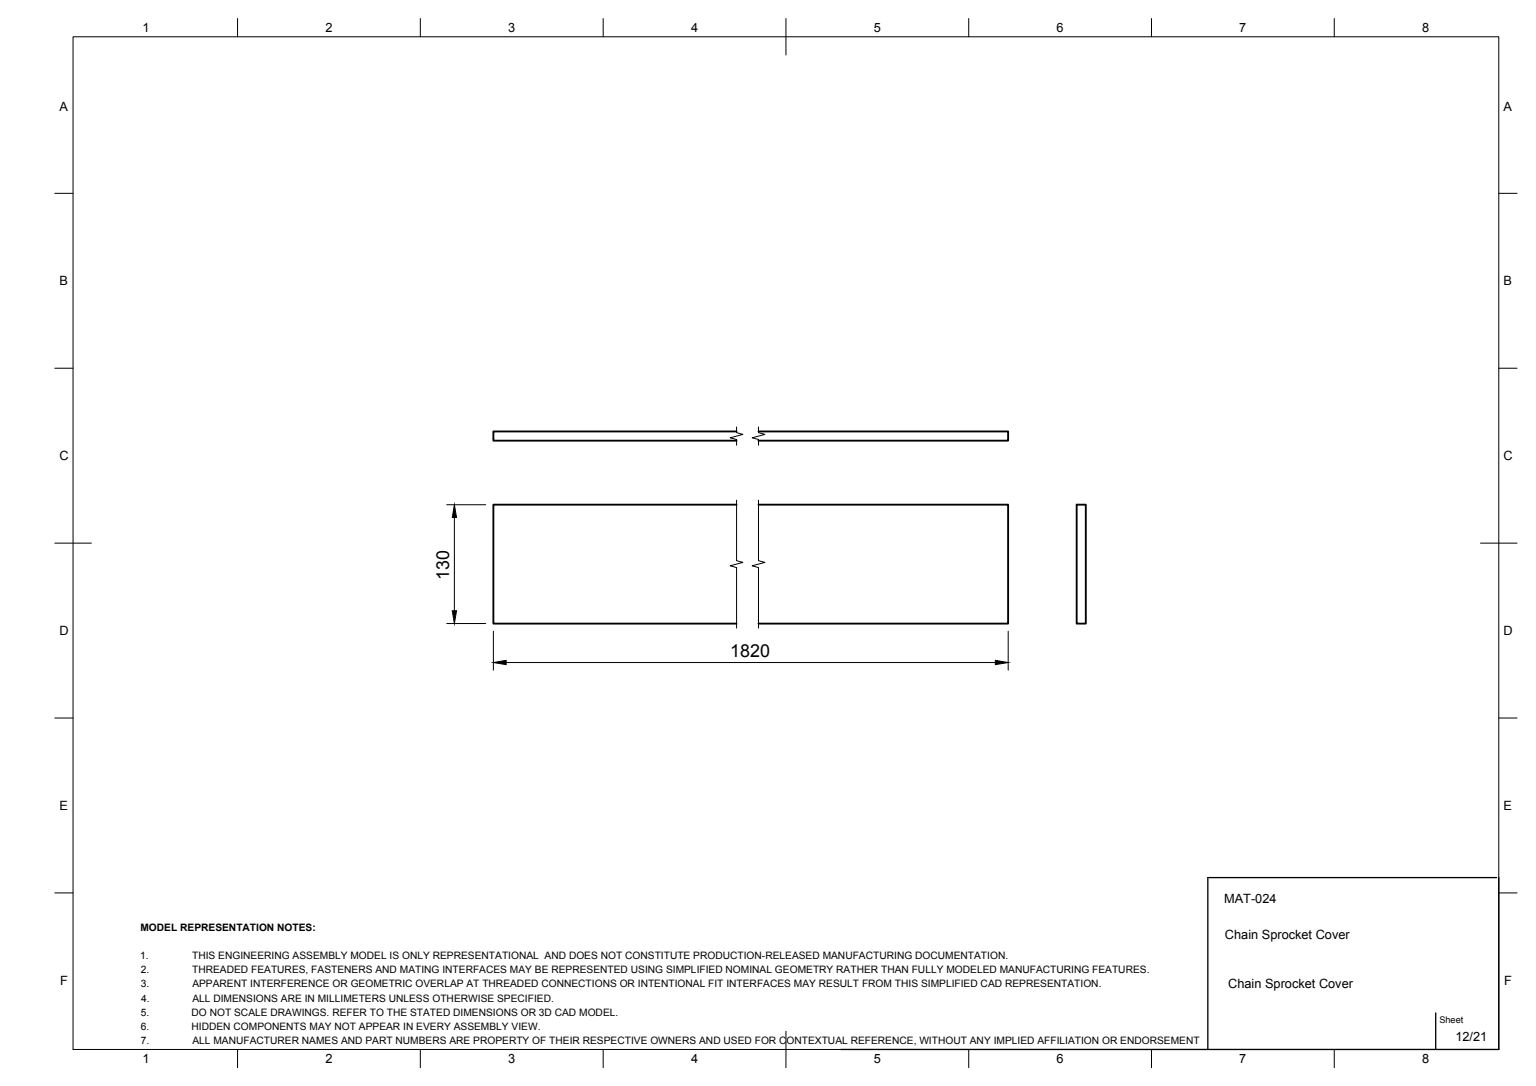
ISO-10303-21;
HEADER;
/* Generated by software containing ST-Developer
 * from STEP Tools, Inc. (www.steptools.com) 
 */

FILE_DESCRIPTION(
/* description */ ('STEP AP214'),
/* implementation_level */ '2;1');

FILE_NAME(
/* name */ 'Chain Sprocket Cover.step',
/* time_stamp */ '2026-11-14T06:34:07-08:00',
/* author */ (''),
/* organization */ (''),
/* preprocessor_version */ 'ST-DEVELOPER v20.2',
/* originating_system */ 'Autodesk Translation Framework v15.17.0.0',
/* authorisation */ '');

FILE_SCHEMA (('AUTOMOTIVE_DESIGN { 1 0 10303 214 3 1 1 }'));
ENDSEC;

DATA;
#10=MECHANICAL_DESIGN_GEOMETRIC_PRESENTATION_REPRESENTATION('',(#7278),#310623);
#7225=SHAPE_REPRESENTATION_RELATIONSHIP('SRR','None',#310897,#7242);
#7242=ADVANCED_BREP_SHAPE_REPRESENTATION('',(#7346),#310606);
#7278=STYLED_ITEM('',(#311006),#7346);
#7346=MANIFOLD_SOLID_BREP('Body1',#93728);
#8518=PLANE('',#103333);
#8519=PLANE('',#103334);
#8520=PLANE('',#103335);
#8521=PLANE('',#103336);
#8522=PLANE('',#103337);
#8523=PLANE('',#103338);
#13629=FACE_OUTER_BOUND('',#19599,.T.);
#13630=FACE_OUTER_BOUND('',#19600,.T.);
#13631=FACE_OUTER_BOUND('',#19601,.T.);
#13632=FACE_OUTER_BOUND('',#19602,.T.);
#13633=FACE_OUTER_BOUND('',#19603,.T.);
#13634=FACE_OUTER_BOUND('',#19604,.T.);
#19599=EDGE_LOOP('',(#81693,#81694,#81695,#81696));
#19600=EDGE_LOOP('',(#81697,#81698,#81699,#81700));
#19601=EDGE_LOOP('',(#81701,#81702,#81703,#81704));
#19602=EDGE_LOOP('',(#81705,#81706,#81707,#81708));
#19603=EDGE_LOOP('',(#81709,#81710,#81711,#81712));
#19604=EDGE_LOOP('',(#81713,#81714,#81715,#81716));
#24192=LINE('',#271199,#28539);
#24193=LINE('',#271201,#28540);
#24194=LINE('',#271203,#28541);
#24195=LINE('',#271204,#28542);
#24196=LINE('',#271207,#28543);
#24197=LINE('',#271209,#28544);
#24198=LINE('',#271210,#28545);
#24199=LINE('',#271213,#28546);
#24200=LINE('',#271215,#28547);
#24201=LINE('',#271216,#28548);
#24202=LINE('',#271218,#28549);
#24203=LINE('',#271219,#28550);
#28539=VECTOR('',#127317,1000.);
#28540=VECTOR('',#127318,1000.);
#28541=VECTOR('',#127319,1000.);
#28542=VECTOR('',#127320,1000.);
#28543=VECTOR('',#127323,1000.);
#28544=VECTOR('',#127324,1000.);
#28545=VECTOR('',#127325,1000.);
#28546=VECTOR('',#127328,1000.);
#28547=VECTOR('',#127329,1000.);
#28548=VECTOR('',#127330,1000.);
#28549=VECTOR('',#127333,1000.);
#28550=VECTOR('',#127334,1000.);
#42245=VERTEX_POINT('',#271197);
#42246=VERTEX_POINT('',#271198);
#42247=VERTEX_POINT('',#271200);
#42248=VERTEX_POINT('',#271202);
#42249=VERTEX_POINT('',#271206);
#42250=VERTEX_POINT('',#271208);
#42251=VERTEX_POINT('',#271212);
#42252=VERTEX_POINT('',#271214);
#55626=EDGE_CURVE('',#42245,#42246,#24192,.T.);
#55627=EDGE_CURVE('',#42247,#42246,#24193,.T.);
#55628=EDGE_CURVE('',#42248,#42247,#24194,.T.);
#55629=EDGE_CURVE('',#42248,#42245,#24195,.T.);
#55630=EDGE_CURVE('',#42246,#42249,#24196,.T.);
#55631=EDGE_CURVE('',#42250,#42249,#24197,.T.);
#55632=EDGE_CURVE('',#42247,#42250,#24198,.T.);
#55633=EDGE_CURVE('',#42249,#42251,#24199,.T.);
#55634=EDGE_CURVE('',#42252,#42251,#24200,.T.);
#55635=EDGE_CURVE('',#42250,#42252,#24201,.T.);
#55636=EDGE_CURVE('',#42251,#42245,#24202,.T.);
#55637=EDGE_CURVE('',#42252,#42248,#24203,.T.);
#81693=ORIENTED_EDGE('',*,*,#55626,.T.);
#81694=ORIENTED_EDGE('',*,*,#55627,.F.);
#81695=ORIENTED_EDGE('',*,*,#55628,.F.);
#81696=ORIENTED_EDGE('',*,*,#55629,.T.);
#81697=ORIENTED_EDGE('',*,*,#55630,.T.);
#81698=ORIENTED_EDGE('',*,*,#55631,.F.);
#81699=ORIENTED_EDGE('',*,*,#55632,.F.);
#81700=ORIENTED_EDGE('',*,*,#55627,.T.);
#81701=ORIENTED_EDGE('',*,*,#55633,.T.);
#81702=ORIENTED_EDGE('',*,*,#55634,.F.);
#81703=ORIENTED_EDGE('',*,*,#55635,.F.);
#81704=ORIENTED_EDGE('',*,*,#55631,.T.);
#81705=ORIENTED_EDGE('',*,*,#55636,.T.);
#81706=ORIENTED_EDGE('',*,*,#55629,.F.);
#81707=ORIENTED_EDGE('',*,*,#55637,.F.);
#81708=ORIENTED_EDGE('',*,*,#55634,.T.);
#81709=ORIENTED_EDGE('',*,*,#55628,.T.);
#81710=ORIENTED_EDGE('',*,*,#55632,.T.);
#81711=ORIENTED_EDGE('',*,*,#55635,.T.);
#81712=ORIENTED_EDGE('',*,*,#55637,.T.);
#81713=ORIENTED_EDGE('',*,*,#55626,.F.);
#81714=ORIENTED_EDGE('',*,*,#55636,.F.);
#81715=ORIENTED_EDGE('',*,*,#55633,.F.);
#81716=ORIENTED_EDGE('',*,*,#55630,.F.);
#92908=ADVANCED_FACE('',(#13629),#8518,.F.);
#92909=ADVANCED_FACE('',(#13630),#8519,.F.);
#92910=ADVANCED_FACE('',(#13631),#8520,.F.);
#92911=ADVANCED_FACE('',(#13632),#8521,.F.);
#92912=ADVANCED_FACE('',(#13633),#8522,.T.);
#92913=ADVANCED_FACE('',(#13634),#8523,.F.);
#93728=CLOSED_SHELL('',(#92908,#92909,#92910,#92911,#92912,#92913));
#103332=AXIS2_PLACEMENT_3D('',#271195,#127313,#127314);
#103333=AXIS2_PLACEMENT_3D('',#271196,#127315,#127316);
#103334=AXIS2_PLACEMENT_3D('',#271205,#127321,#127322);
#103335=AXIS2_PLACEMENT_3D('',#271211,#127326,#127327);
#103336=AXIS2_PLACEMENT_3D('',#271217,#127331,#127332);
#103337=AXIS2_PLACEMENT_3D('',#271220,#127335,#127336);
#103338=AXIS2_PLACEMENT_3D('',#271221,#127337,#127338);
#127313=DIRECTION('axis',(0.,0.,1.));
#127314=DIRECTION('refdir',(1.,0.,0.));
#127315=DIRECTION('center_axis',(0.,0.,-1.));
#127316=DIRECTION('ref_axis',(-1.,0.,0.));
#127317=DIRECTION('',(0.,-1.,0.));
#127318=DIRECTION('',(-1.,0.,0.));
#127319=DIRECTION('',(0.,-1.,0.));
#127320=DIRECTION('',(-1.,0.,0.));
#127321=DIRECTION('center_axis',(0.,1.,1.52503162723236E-17));
#127322=DIRECTION('ref_axis',(0.,-1.52503162723236E-17,1.));
#127323=DIRECTION('',(0.,1.52503162723236E-17,-1.));
#127324=DIRECTION('',(-1.,0.,0.));
#127325=DIRECTION('',(0.,1.52503162723236E-17,-1.));
#127326=DIRECTION('center_axis',(0.,0.,1.));
#127327=DIRECTION('ref_axis',(1.,0.,0.));
#127328=DIRECTION('',(0.,1.,0.));
#127329=DIRECTION('',(-1.,0.,0.));
#127330=DIRECTION('',(0.,1.,0.));
#127331=DIRECTION('center_axis',(0.,-1.,0.));
#127332=DIRECTION('ref_axis',(0.,0.,-1.));
#127333=DIRECTION('',(0.,0.,1.));
#127334=DIRECTION('',(0.,0.,1.));
#127335=DIRECTION('center_axis',(1.,0.,0.));
#127336=DIRECTION('ref_axis',(0.,0.,-1.));
#127337=DIRECTION('center_axis',(1.,0.,0.));
#127338=DIRECTION('ref_axis',(0.,0.,-1.));
#271195=CARTESIAN_POINT('',(0.,0.,0.));
#271196=CARTESIAN_POINT('Origin',(10.,130.,910.));
#271197=CARTESIAN_POINT('',(0.,130.,910.));
#271198=CARTESIAN_POINT('',(0.,0.,910.));
#271199=CARTESIAN_POINT('',(0.,130.,910.));
#271200=CARTESIAN_POINT('',(10.,0.,910.));
#271201=CARTESIAN_POINT('',(10.,0.,910.));
#271202=CARTESIAN_POINT('',(10.,130.,910.));
#271203=CARTESIAN_POINT('',(10.,130.,910.));
#271204=CARTESIAN_POINT('',(10.,130.,910.));
#271205=CARTESIAN_POINT('Origin',(10.,0.,910.));
#271206=CARTESIAN_POINT('',(0.,2.77555756156289E-14,-910.));
#271207=CARTESIAN_POINT('',(0.,0.,910.));
#271208=CARTESIAN_POINT('',(10.,2.77555756156289E-14,-910.));
#271209=CARTESIAN_POINT('',(10.,2.77555756156289E-14,-910.));
#271210=CARTESIAN_POINT('',(10.,0.,910.));
#271211=CARTESIAN_POINT('Origin',(10.,130.,-910.));
#271212=CARTESIAN_POINT('',(0.,130.,-910.));
#271213=CARTESIAN_POINT('',(0.,130.,-910.));
#271214=CARTESIAN_POINT('',(10.,130.,-910.));
#271215=CARTESIAN_POINT('',(10.,130.,-910.));
#271216=CARTESIAN_POINT('',(10.,130.,-910.));
#271217=CARTESIAN_POINT('Origin',(10.,130.,910.));
#271218=CARTESIAN_POINT('',(0.,130.,910.));
#271219=CARTESIAN_POINT('',(10.,130.,910.));
#271220=CARTESIAN_POINT('Origin',(10.,0.,0.));
#271221=CARTESIAN_POINT('Origin',(0.,0.,0.));
#310584=UNCERTAINTY_MEASURE_WITH_UNIT(LENGTH_MEASURE(0.01),#310624,
'DISTANCE_ACCURACY_VALUE',
'Maximum model space distance between geometric entities at asserted c
onnectivities');
#310601=UNCERTAINTY_MEASURE_WITH_UNIT(LENGTH_MEASURE(0.01),#310624,
'DISTANCE_ACCURACY_VALUE',
'Maximum model space distance between geometric entities at asserted c
onnectivities');
#310606=(
GEOMETRIC_REPRESENTATION_CONTEXT(3)
GLOBAL_UNCERTAINTY_ASSIGNED_CONTEXT((#310584))
GLOBAL_UNIT_ASSIGNED_CONTEXT((#310624,#310626,#310627))
REPRESENTATION_CONTEXT('','3D')
);
#310623=(
GEOMETRIC_REPRESENTATION_CONTEXT(3)
GLOBAL_UNCERTAINTY_ASSIGNED_CONTEXT((#310601))
GLOBAL_UNIT_ASSIGNED_CONTEXT((#310624,#310626,#310627))
REPRESENTATION_CONTEXT('','3D')
);
#310624=(
LENGTH_UNIT()
NAMED_UNIT(*)
SI_UNIT(.MILLI.,.METRE.)
);
#310626=(
NAMED_UNIT(*)
PLANE_ANGLE_UNIT()
SI_UNIT($,.RADIAN.)
);
#310627=(
NAMED_UNIT(*)
SI_UNIT($,.STERADIAN.)
SOLID_ANGLE_UNIT()
);
#310632=SHAPE_DEFINITION_REPRESENTATION(#310653,#310897);
#310653=PRODUCT_DEFINITION_SHAPE('',$,#310919);
#310897=SHAPE_REPRESENTATION('',(#103332),#310606);
#310914=PRODUCT_DEFINITION_CONTEXT('part definition',#310979,'design');
#310919=PRODUCT_DEFINITION('Chain Sprocket Cover',
'Chain Sprocket Cover',#310940,#310914);
#310940=PRODUCT_DEFINITION_FORMATION('',$,#310985);
#310979=APPLICATION_CONTEXT(
'Core Data for Automotive Mechanical Design Process');
#310980=PRODUCT_CONTEXT('part definition',#310979,'mechanical');
#310985=PRODUCT('Chain Sprocket Cover','Chain Sprocket Cover',$,(#310980));
#311006=PRESENTATION_STYLE_ASSIGNMENT((#311013));
#311013=SURFACE_STYLE_USAGE(.BOTH.,#311020);
#311020=SURFACE_SIDE_STYLE('',(#311027));
#311027=SURFACE_STYLE_FILL_AREA(#311034);
#311034=FILL_AREA_STYLE('Opaque(61,176,222)',(#311041));
#311041=FILL_AREA_STYLE_COLOUR('Opaque(61,176,222)',#311048);
#311048=COLOUR_RGB('Opaque(61,176,222)',0.23921568627451,0.690196078431373,
0.870588235294118);
ENDSEC;
END-ISO-10303-21;
